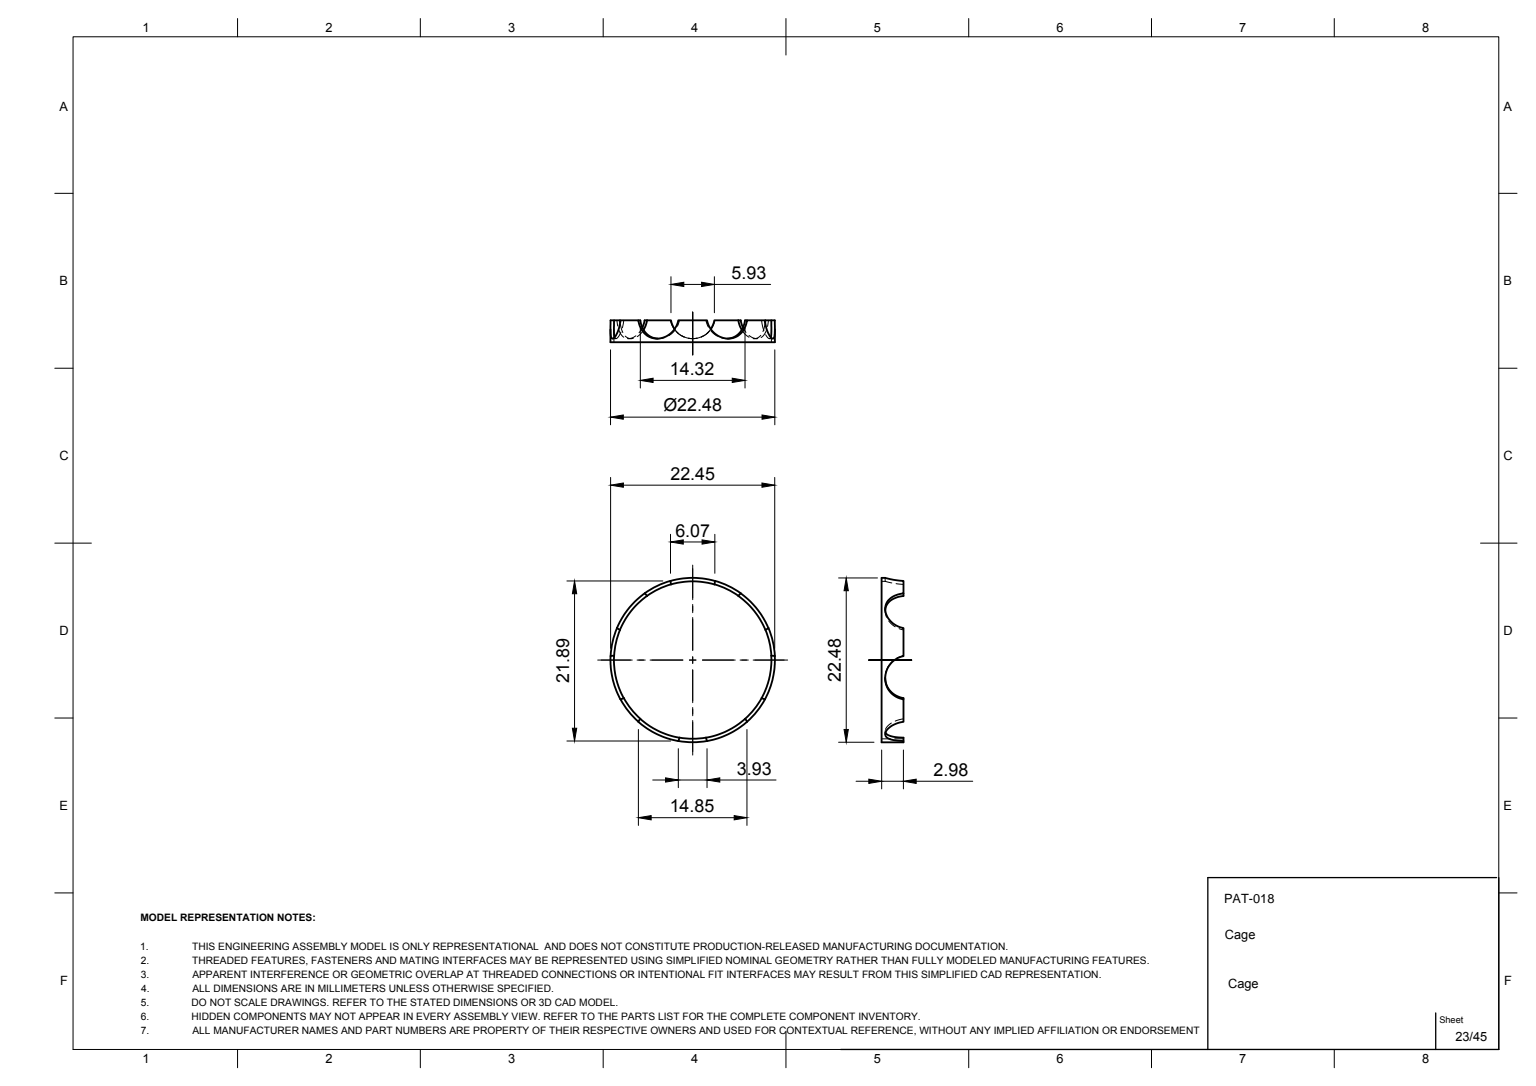
ISO-10303-21;
HEADER;
/* Generated by software containing ST-Developer
 * from STEP Tools, Inc. (www.steptools.com) 
 */

FILE_DESCRIPTION(
/* description */ ('Cam-driven reciprocating slide'),
/* implementation_level */ '2;1');

FILE_NAME(
/* name */ 'Cage.step',
/* time_stamp */ '2026-10-28T03:25:20-07:00',
/* author */ (''),
/* organization */ (''),
/* preprocessor_version */ 'ST-DEVELOPER v20.2',
/* originating_system */ 'Autodesk Translation Framework v15.17.0.0',
/* authorisation */ '');

FILE_SCHEMA (('AUTOMOTIVE_DESIGN { 1 0 10303 214 3 1 1 }'));
ENDSEC;

DATA;
#10=MECHANICAL_DESIGN_GEOMETRIC_PRESENTATION_REPRESENTATION('',(#444),#13277);
#308=SPHERICAL_SURFACE('',#7211,0.309556);
#309=SPHERICAL_SURFACE('',#7227,0.309556);
#310=SPHERICAL_SURFACE('',#7232,0.309556);
#311=SPHERICAL_SURFACE('',#7238,0.309556);
#312=SPHERICAL_SURFACE('',#7243,0.309556);
#313=SPHERICAL_SURFACE('',#7248,0.309556);
#314=SPHERICAL_SURFACE('',#7256,0.309556);
#333=B_SPLINE_CURVE_WITH_KNOTS('',3,(#11932,#11933,#11934,#11935,#11936,
#11937,#11938,#11939,#11940,#11941,#11942,#11943,#11944,#11945,#11946,#11947,
#11948,#11949,#11950,#11951,#11952,#11953),.UNSPECIFIED.,.F.,.F.,(4,2,2,
2,2,2,2,2,2,2,4),(0.0591825211272536,0.157966726598481,0.236950089897721,
0.315933453196962,0.391576304923761,0.46721915665056,0.54286200837736,0.618504860104159,
0.697488223403399,0.77647158670264,0.875255792173867),.UNSPECIFIED.);
#334=B_SPLINE_CURVE_WITH_KNOTS('',3,(#11957,#11958,#11959,#11960,#11961,
#11962,#11963,#11964,#11965,#11966,#11967,#11968,#11969,#11970,#11971,#11972,
#11973,#11974,#11975,#11976,#11977,#11978),.UNSPECIFIED.,.F.,.F.,(4,2,2,
2,2,2,2,2,2,2,4),(0.0581119756758434,0.106553146291161,0.213106292582322,
0.30849933801665,0.386091982889075,0.4636846277615,0.541277272633925,0.61886991750635,
0.714262962940678,0.820816109231839,0.869257279847157),.UNSPECIFIED.);
#335=B_SPLINE_CURVE_WITH_KNOTS('',3,(#11984,#11985,#11986,#11987,#11988,
#11989,#11990,#11991,#11992,#11993,#11994,#11995,#11996,#11997,#11998,#11999,
#12000,#12001,#12002,#12003,#12004,#12005),.UNSPECIFIED.,.F.,.F.,(4,2,2,
2,2,2,2,2,2,2,4),(0.0581119756758434,0.106553146291161,0.213106292582322,
0.30849933801665,0.386091982889075,0.4636846277615,0.541277272633925,0.61886991750635,
0.714262962940679,0.820816109231839,0.869257279847157),.UNSPECIFIED.);
#336=B_SPLINE_CURVE_WITH_KNOTS('',3,(#12009,#12010,#12011,#12012,#12013,
#12014,#12015,#12016,#12017,#12018,#12019,#12020,#12021,#12022,#12023,#12024,
#12025,#12026,#12027,#12028,#12029,#12030),.UNSPECIFIED.,.F.,.F.,(4,2,2,
2,2,2,2,2,2,2,4),(0.0581119756758433,0.106553146291161,0.213106292582322,
0.308499338016649,0.386091982889075,0.4636846277615,0.541277272633925,0.61886991750635,
0.714262962940678,0.820816109231839,0.869257279847157),.UNSPECIFIED.);
#337=B_SPLINE_CURVE_WITH_KNOTS('',3,(#12039,#12040,#12041,#12042,#12043,
#12044,#12045,#12046,#12047,#12048,#12049,#12050,#12051,#12052,#12053,#12054,
#12055,#12056,#12057,#12058,#12059,#12060),.UNSPECIFIED.,.F.,.F.,(4,2,2,
2,2,2,2,2,2,2,4),(0.0581119756758433,0.106553146291161,0.213106292582322,
0.30849933801665,0.386091982889075,0.4636846277615,0.541277272633925,0.61886991750635,
0.714262962940678,0.820816109231839,0.869257279847157),.UNSPECIFIED.);
#338=B_SPLINE_CURVE_WITH_KNOTS('',3,(#12064,#12065,#12066,#12067,#12068,
#12069,#12070,#12071,#12072,#12073,#12074,#12075,#12076,#12077,#12078,#12079,
#12080,#12081,#12082,#12083,#12084,#12085),.UNSPECIFIED.,.F.,.F.,(4,2,2,
2,2,2,2,2,2,2,4),(0.0581119756758434,0.106553146291161,0.213106292582322,
0.30849933801665,0.386091982889075,0.4636846277615,0.541277272633925,0.61886991750635,
0.714262962940678,0.820816109231839,0.869257279847157),.UNSPECIFIED.);
#339=B_SPLINE_CURVE_WITH_KNOTS('',3,(#12089,#12090,#12091,#12092,#12093,
#12094,#12095,#12096,#12097,#12098,#12099,#12100,#12101,#12102,#12103,#12104,
#12105,#12106,#12107,#12108,#12109,#12110),.UNSPECIFIED.,.F.,.F.,(4,2,2,
2,2,2,2,2,2,2,4),(0.0581119756758434,0.106553146291161,0.213106292582322,
0.30849933801665,0.386091982889075,0.4636846277615,0.541277272633925,0.61886991750635,
0.714262962940678,0.820816109231839,0.869257279847157),.UNSPECIFIED.);
#340=B_SPLINE_CURVE_WITH_KNOTS('',3,(#12114,#12115,#12116,#12117,#12118,
#12119,#12120,#12121,#12122,#12123,#12124,#12125,#12126,#12127,#12128,#12129,
#12130,#12131,#12132,#12133,#12134,#12135),.UNSPECIFIED.,.F.,.F.,(4,2,2,
2,2,2,2,2,2,2,4),(0.0581119756758433,0.106553146291161,0.213106292582322,
0.30849933801665,0.386091982889075,0.4636846277615,0.541277272633925,0.61886991750635,
0.714262962940678,0.820816109231839,0.869257279847157),.UNSPECIFIED.);
#341=B_SPLINE_CURVE_WITH_KNOTS('',3,(#12143,#12144,#12145,#12146,#12147,
#12148,#12149,#12150,#12151,#12152,#12153,#12154,#12155,#12156,#12157,#12158,
#12159,#12160,#12161,#12162,#12163,#12164),.UNSPECIFIED.,.F.,.F.,(4,2,2,
2,2,2,2,2,2,2,4),(0.0591825211272536,0.157966726598481,0.236950089897721,
0.315933453196962,0.391576304923761,0.467219156650561,0.54286200837736,
0.618504860104159,0.697488223403399,0.77647158670264,0.875255792173867),
 .UNSPECIFIED.);
#342=B_SPLINE_CURVE_WITH_KNOTS('',3,(#12172,#12173,#12174,#12175,#12176,
#12177,#12178,#12179,#12180,#12181,#12182,#12183,#12184,#12185,#12186,#12187,
#12188,#12189,#12190,#12191,#12192,#12193),.UNSPECIFIED.,.F.,.F.,(4,2,2,
2,2,2,2,2,2,2,4),(0.0591825211272536,0.157966726598481,0.236950089897722,
0.315933453196962,0.391576304923761,0.467219156650561,0.54286200837736,
0.618504860104159,0.697488223403399,0.77647158670264,0.875255792173867),
 .UNSPECIFIED.);
#343=B_SPLINE_CURVE_WITH_KNOTS('',3,(#12203,#12204,#12205,#12206,#12207,
#12208,#12209,#12210,#12211,#12212,#12213,#12214,#12215,#12216,#12217,#12218,
#12219,#12220,#12221,#12222,#12223,#12224),.UNSPECIFIED.,.F.,.F.,(4,2,2,
2,2,2,2,2,2,2,4),(0.0591825211272536,0.157966726598481,0.236950089897721,
0.315933453196962,0.391576304923761,0.46721915665056,0.54286200837736,0.618504860104159,
0.697488223403399,0.77647158670264,0.875255792173867),.UNSPECIFIED.);
#344=B_SPLINE_CURVE_WITH_KNOTS('',3,(#12232,#12233,#12234,#12235,#12236,
#12237,#12238,#12239,#12240,#12241,#12242,#12243,#12244,#12245,#12246,#12247,
#12248,#12249,#12250,#12251,#12252,#12253),.UNSPECIFIED.,.F.,.F.,(4,2,2,
2,2,2,2,2,2,2,4),(0.0591825211272536,0.157966726598481,0.236950089897721,
0.315933453196962,0.391576304923761,0.46721915665056,0.542862008377359,
0.618504860104159,0.697488223403399,0.776471586702639,0.875255792173867),
 .UNSPECIFIED.);
#345=B_SPLINE_CURVE_WITH_KNOTS('',3,(#12261,#12262,#12263,#12264,#12265,
#12266,#12267,#12268,#12269,#12270,#12271,#12272,#12273,#12274,#12275,#12276,
#12277,#12278,#12279,#12280,#12281,#12282),.UNSPECIFIED.,.F.,.F.,(4,2,2,
2,2,2,2,2,2,2,4),(0.0591825211272536,0.157966726598481,0.236950089897721,
0.315933453196962,0.391576304923761,0.46721915665056,0.54286200837736,0.618504860104159,
0.697488223403399,0.77647158670264,0.875255792173867),.UNSPECIFIED.);
#346=B_SPLINE_CURVE_WITH_KNOTS('',3,(#12291,#12292,#12293,#12294,#12295,
#12296,#12297,#12298,#12299,#12300,#12301,#12302,#12303,#12304,#12305,#12306,
#12307,#12308,#12309,#12310,#12311,#12312),.UNSPECIFIED.,.F.,.F.,(4,2,2,
2,2,2,2,2,2,2,4),(0.0591825211272536,0.157966726598481,0.236950089897721,
0.315933453196962,0.391576304923761,0.46721915665056,0.542862008377359,
0.618504860104159,0.697488223403399,0.776471586702639,0.875255792173867),
 .UNSPECIFIED.);
#364=SHAPE_REPRESENTATION_RELATIONSHIP('SRR','None',#13458,#401);
#401=ADVANCED_BREP_SHAPE_REPRESENTATION('',(#488),#13253);
#444=STYLED_ITEM('',(#13720),#488);
#488=MANIFOLD_SOLID_BREP('Continuous crown cage',#6420);
#622=FACE_BOUND('',#1585,.T.);
#768=PLANE('',#7224);
#769=PLANE('',#7229);
#770=PLANE('',#7234);
#771=PLANE('',#7240);
#772=PLANE('',#7245);
#773=PLANE('',#7254);
#774=PLANE('',#7258);
#775=PLANE('',#7259);
#1075=FACE_OUTER_BOUND('',#1569,.T.);
#1076=FACE_OUTER_BOUND('',#1570,.T.);
#1077=FACE_OUTER_BOUND('',#1571,.T.);
#1078=FACE_OUTER_BOUND('',#1572,.T.);
#1079=FACE_OUTER_BOUND('',#1573,.T.);
#1080=FACE_OUTER_BOUND('',#1574,.T.);
#1081=FACE_OUTER_BOUND('',#1575,.T.);
#1082=FACE_OUTER_BOUND('',#1576,.T.);
#1083=FACE_OUTER_BOUND('',#1577,.T.);
#1084=FACE_OUTER_BOUND('',#1578,.T.);
#1085=FACE_OUTER_BOUND('',#1579,.T.);
#1086=FACE_OUTER_BOUND('',#1580,.T.);
#1087=FACE_OUTER_BOUND('',#1581,.T.);
#1088=FACE_OUTER_BOUND('',#1582,.T.);
#1089=FACE_OUTER_BOUND('',#1583,.T.);
#1090=FACE_OUTER_BOUND('',#1584,.T.);
#1091=FACE_OUTER_BOUND('',#1586,.T.);
#1569=EDGE_LOOP('',(#5086,#5087,#5088,#5089));
#1570=EDGE_LOOP('',(#5090,#5091,#5092,#5093,#5094,#5095,#5096,#5097,#5098,
#5099,#5100,#5101,#5102,#5103,#5104,#5105,#5106,#5107));
#1571=EDGE_LOOP('',(#5108,#5109,#5110,#5111));
#1572=EDGE_LOOP('',(#5112,#5113,#5114,#5115));
#1573=EDGE_LOOP('',(#5116,#5117,#5118,#5119));
#1574=EDGE_LOOP('',(#5120,#5121,#5122,#5123));
#1575=EDGE_LOOP('',(#5124,#5125,#5126,#5127,#5128,#5129));
#1576=EDGE_LOOP('',(#5130,#5131,#5132,#5133));
#1577=EDGE_LOOP('',(#5134,#5135,#5136,#5137));
#1578=EDGE_LOOP('',(#5138,#5139,#5140,#5141));
#1579=EDGE_LOOP('',(#5142,#5143,#5144,#5145));
#1580=EDGE_LOOP('',(#5146,#5147,#5148,#5149));
#1581=EDGE_LOOP('',(#5150,#5151,#5152,#5153,#5154,#5155,#5156,#5157,#5158,
#5159,#5160,#5161,#5162,#5163,#5164,#5165,#5166,#5167));
#1582=EDGE_LOOP('',(#5168,#5169,#5170,#5171));
#1583=EDGE_LOOP('',(#5172,#5173,#5174,#5175));
#1584=EDGE_LOOP('',(#5176));
#1585=EDGE_LOOP('',(#5177));
#1586=EDGE_LOOP('',(#5178,#5179,#5180,#5181));
#2042=LINE('',#12034,#2481);
#2043=LINE('',#12287,#2482);
#2481=VECTOR('',#8608,1.123812);
#2482=VECTOR('',#8677,1.076188);
#2876=CIRCLE('',#7212,0.303778037777585);
#2877=CIRCLE('',#7213,0.303778037777585);
#2878=CIRCLE('',#7215,1.123812);
#2879=CIRCLE('',#7216,1.123812);
#2880=CIRCLE('',#7217,1.123812);
#2881=CIRCLE('',#7218,1.123812);
#2882=CIRCLE('',#7219,1.123812);
#2883=CIRCLE('',#7220,1.123812);
#2884=CIRCLE('',#7221,1.123812);
#2885=CIRCLE('',#7222,1.123812);
#2886=CIRCLE('',#7223,1.123812);
#2887=CIRCLE('',#7225,1.076188);
#2888=CIRCLE('',#7226,0.303778037777585);
#2889=CIRCLE('',#7228,0.303778037777585);
#2890=CIRCLE('',#7230,1.076188);
#2891=CIRCLE('',#7231,0.303778037777585);
#2892=CIRCLE('',#7233,0.303778037777585);
#2893=CIRCLE('',#7235,1.076188);
#2894=CIRCLE('',#7236,1.076188);
#2895=CIRCLE('',#7237,0.303778037777585);
#2896=CIRCLE('',#7239,0.303778037777585);
#2897=CIRCLE('',#7241,1.076188);
#2898=CIRCLE('',#7242,0.303778037777585);
#2899=CIRCLE('',#7244,0.303778037777585);
#2900=CIRCLE('',#7246,1.076188);
#2901=CIRCLE('',#7247,0.303778037777585);
#2902=CIRCLE('',#7249,0.303778037777585);
#2903=CIRCLE('',#7251,1.076188);
#2904=CIRCLE('',#7252,1.076188);
#2905=CIRCLE('',#7253,1.076188);
#2906=CIRCLE('',#7255,0.303778037777585);
#2907=CIRCLE('',#7257,0.303778037777585);
#3293=VERTEX_POINT('',#11930);
#3294=VERTEX_POINT('',#11931);
#3295=VERTEX_POINT('',#11954);
#3296=VERTEX_POINT('',#11956);
#3297=VERTEX_POINT('',#11981);
#3298=VERTEX_POINT('',#11983);
#3299=VERTEX_POINT('',#12006);
#3300=VERTEX_POINT('',#12008);
#3301=VERTEX_POINT('',#12031);
#3302=VERTEX_POINT('',#12033);
#3303=VERTEX_POINT('',#12036);
#3304=VERTEX_POINT('',#12038);
#3305=VERTEX_POINT('',#12061);
#3306=VERTEX_POINT('',#12063);
#3307=VERTEX_POINT('',#12086);
#3308=VERTEX_POINT('',#12088);
#3309=VERTEX_POINT('',#12111);
#3310=VERTEX_POINT('',#12113);
#3311=VERTEX_POINT('',#12138);
#3312=VERTEX_POINT('',#12142);
#3313=VERTEX_POINT('',#12167);
#3314=VERTEX_POINT('',#12171);
#3315=VERTEX_POINT('',#12196);
#3316=VERTEX_POINT('',#12198);
#3317=VERTEX_POINT('',#12202);
#3318=VERTEX_POINT('',#12227);
#3319=VERTEX_POINT('',#12231);
#3320=VERTEX_POINT('',#12256);
#3321=VERTEX_POINT('',#12260);
#3322=VERTEX_POINT('',#12285);
#3323=VERTEX_POINT('',#12288);
#3324=VERTEX_POINT('',#12290);
#3933=EDGE_CURVE('',#3293,#3294,#333,.T.);
#3934=EDGE_CURVE('',#3295,#3293,#2876,.T.);
#3935=EDGE_CURVE('',#3296,#3295,#334,.T.);
#3936=EDGE_CURVE('',#3294,#3296,#2877,.T.);
#3937=EDGE_CURVE('',#3297,#3295,#2878,.T.);
#3938=EDGE_CURVE('',#3297,#3298,#335,.T.);
#3939=EDGE_CURVE('',#3299,#3298,#2879,.T.);
#3940=EDGE_CURVE('',#3299,#3300,#336,.T.);
#3941=EDGE_CURVE('',#3301,#3300,#2880,.T.);
#3942=EDGE_CURVE('',#3301,#3302,#2042,.T.);
#3943=EDGE_CURVE('',#3302,#3302,#2881,.T.);
#3944=EDGE_CURVE('',#3303,#3301,#2882,.T.);
#3945=EDGE_CURVE('',#3303,#3304,#337,.T.);
#3946=EDGE_CURVE('',#3305,#3304,#2883,.T.);
#3947=EDGE_CURVE('',#3305,#3306,#338,.T.);
#3948=EDGE_CURVE('',#3307,#3306,#2884,.T.);
#3949=EDGE_CURVE('',#3307,#3308,#339,.T.);
#3950=EDGE_CURVE('',#3309,#3308,#2885,.T.);
#3951=EDGE_CURVE('',#3309,#3310,#340,.T.);
#3952=EDGE_CURVE('',#3296,#3310,#2886,.T.);
#3953=EDGE_CURVE('',#3293,#3311,#2887,.T.);
#3954=EDGE_CURVE('',#3311,#3297,#2888,.T.);
#3955=EDGE_CURVE('',#3312,#3311,#341,.T.);
#3956=EDGE_CURVE('',#3298,#3312,#2889,.T.);
#3957=EDGE_CURVE('',#3312,#3313,#2890,.T.);
#3958=EDGE_CURVE('',#3313,#3299,#2891,.T.);
#3959=EDGE_CURVE('',#3314,#3313,#342,.T.);
#3960=EDGE_CURVE('',#3300,#3314,#2892,.T.);
#3961=EDGE_CURVE('',#3314,#3315,#2893,.T.);
#3962=EDGE_CURVE('',#3315,#3316,#2894,.T.);
#3963=EDGE_CURVE('',#3316,#3303,#2895,.T.);
#3964=EDGE_CURVE('',#3317,#3316,#343,.T.);
#3965=EDGE_CURVE('',#3304,#3317,#2896,.T.);
#3966=EDGE_CURVE('',#3317,#3318,#2897,.T.);
#3967=EDGE_CURVE('',#3318,#3305,#2898,.T.);
#3968=EDGE_CURVE('',#3319,#3318,#344,.T.);
#3969=EDGE_CURVE('',#3306,#3319,#2899,.T.);
#3970=EDGE_CURVE('',#3319,#3320,#2900,.T.);
#3971=EDGE_CURVE('',#3320,#3307,#2901,.T.);
#3972=EDGE_CURVE('',#3321,#3320,#345,.T.);
#3973=EDGE_CURVE('',#3308,#3321,#2902,.T.);
#3974=EDGE_CURVE('',#3322,#3322,#2903,.T.);
#3975=EDGE_CURVE('',#3322,#3315,#2043,.T.);
#3976=EDGE_CURVE('',#3323,#3294,#2904,.T.);
#3977=EDGE_CURVE('',#3323,#3324,#346,.T.);
#3978=EDGE_CURVE('',#3321,#3324,#2905,.T.);
#3979=EDGE_CURVE('',#3310,#3323,#2906,.T.);
#3980=EDGE_CURVE('',#3324,#3309,#2907,.T.);
#5086=ORIENTED_EDGE('',*,*,#3933,.F.);
#5087=ORIENTED_EDGE('',*,*,#3934,.F.);
#5088=ORIENTED_EDGE('',*,*,#3935,.F.);
#5089=ORIENTED_EDGE('',*,*,#3936,.F.);
#5090=ORIENTED_EDGE('',*,*,#3935,.T.);
#5091=ORIENTED_EDGE('',*,*,#3937,.F.);
#5092=ORIENTED_EDGE('',*,*,#3938,.T.);
#5093=ORIENTED_EDGE('',*,*,#3939,.F.);
#5094=ORIENTED_EDGE('',*,*,#3940,.T.);
#5095=ORIENTED_EDGE('',*,*,#3941,.F.);
#5096=ORIENTED_EDGE('',*,*,#3942,.T.);
#5097=ORIENTED_EDGE('',*,*,#3943,.F.);
#5098=ORIENTED_EDGE('',*,*,#3942,.F.);
#5099=ORIENTED_EDGE('',*,*,#3944,.F.);
#5100=ORIENTED_EDGE('',*,*,#3945,.T.);
#5101=ORIENTED_EDGE('',*,*,#3946,.F.);
#5102=ORIENTED_EDGE('',*,*,#3947,.T.);
#5103=ORIENTED_EDGE('',*,*,#3948,.F.);
#5104=ORIENTED_EDGE('',*,*,#3949,.T.);
#5105=ORIENTED_EDGE('',*,*,#3950,.F.);
#5106=ORIENTED_EDGE('',*,*,#3951,.T.);
#5107=ORIENTED_EDGE('',*,*,#3952,.F.);
#5108=ORIENTED_EDGE('',*,*,#3934,.T.);
#5109=ORIENTED_EDGE('',*,*,#3953,.T.);
#5110=ORIENTED_EDGE('',*,*,#3954,.T.);
#5111=ORIENTED_EDGE('',*,*,#3937,.T.);
#5112=ORIENTED_EDGE('',*,*,#3955,.F.);
#5113=ORIENTED_EDGE('',*,*,#3956,.F.);
#5114=ORIENTED_EDGE('',*,*,#3938,.F.);
#5115=ORIENTED_EDGE('',*,*,#3954,.F.);
#5116=ORIENTED_EDGE('',*,*,#3956,.T.);
#5117=ORIENTED_EDGE('',*,*,#3957,.T.);
#5118=ORIENTED_EDGE('',*,*,#3958,.T.);
#5119=ORIENTED_EDGE('',*,*,#3939,.T.);
#5120=ORIENTED_EDGE('',*,*,#3959,.F.);
#5121=ORIENTED_EDGE('',*,*,#3960,.F.);
#5122=ORIENTED_EDGE('',*,*,#3940,.F.);
#5123=ORIENTED_EDGE('',*,*,#3958,.F.);
#5124=ORIENTED_EDGE('',*,*,#3960,.T.);
#5125=ORIENTED_EDGE('',*,*,#3961,.T.);
#5126=ORIENTED_EDGE('',*,*,#3962,.T.);
#5127=ORIENTED_EDGE('',*,*,#3963,.T.);
#5128=ORIENTED_EDGE('',*,*,#3944,.T.);
#5129=ORIENTED_EDGE('',*,*,#3941,.T.);
#5130=ORIENTED_EDGE('',*,*,#3964,.F.);
#5131=ORIENTED_EDGE('',*,*,#3965,.F.);
#5132=ORIENTED_EDGE('',*,*,#3945,.F.);
#5133=ORIENTED_EDGE('',*,*,#3963,.F.);
#5134=ORIENTED_EDGE('',*,*,#3965,.T.);
#5135=ORIENTED_EDGE('',*,*,#3966,.T.);
#5136=ORIENTED_EDGE('',*,*,#3967,.T.);
#5137=ORIENTED_EDGE('',*,*,#3946,.T.);
#5138=ORIENTED_EDGE('',*,*,#3968,.F.);
#5139=ORIENTED_EDGE('',*,*,#3969,.F.);
#5140=ORIENTED_EDGE('',*,*,#3947,.F.);
#5141=ORIENTED_EDGE('',*,*,#3967,.F.);
#5142=ORIENTED_EDGE('',*,*,#3969,.T.);
#5143=ORIENTED_EDGE('',*,*,#3970,.T.);
#5144=ORIENTED_EDGE('',*,*,#3971,.T.);
#5145=ORIENTED_EDGE('',*,*,#3948,.T.);
#5146=ORIENTED_EDGE('',*,*,#3949,.F.);
#5147=ORIENTED_EDGE('',*,*,#3971,.F.);
#5148=ORIENTED_EDGE('',*,*,#3972,.F.);
#5149=ORIENTED_EDGE('',*,*,#3973,.F.);
#5150=ORIENTED_EDGE('',*,*,#3974,.F.);
#5151=ORIENTED_EDGE('',*,*,#3975,.T.);
#5152=ORIENTED_EDGE('',*,*,#3961,.F.);
#5153=ORIENTED_EDGE('',*,*,#3959,.T.);
#5154=ORIENTED_EDGE('',*,*,#3957,.F.);
#5155=ORIENTED_EDGE('',*,*,#3955,.T.);
#5156=ORIENTED_EDGE('',*,*,#3953,.F.);
#5157=ORIENTED_EDGE('',*,*,#3933,.T.);
#5158=ORIENTED_EDGE('',*,*,#3976,.F.);
#5159=ORIENTED_EDGE('',*,*,#3977,.T.);
#5160=ORIENTED_EDGE('',*,*,#3978,.F.);
#5161=ORIENTED_EDGE('',*,*,#3972,.T.);
#5162=ORIENTED_EDGE('',*,*,#3970,.F.);
#5163=ORIENTED_EDGE('',*,*,#3968,.T.);
#5164=ORIENTED_EDGE('',*,*,#3966,.F.);
#5165=ORIENTED_EDGE('',*,*,#3964,.T.);
#5166=ORIENTED_EDGE('',*,*,#3962,.F.);
#5167=ORIENTED_EDGE('',*,*,#3975,.F.);
#5168=ORIENTED_EDGE('',*,*,#3936,.T.);
#5169=ORIENTED_EDGE('',*,*,#3952,.T.);
#5170=ORIENTED_EDGE('',*,*,#3979,.T.);
#5171=ORIENTED_EDGE('',*,*,#3976,.T.);
#5172=ORIENTED_EDGE('',*,*,#3951,.F.);
#5173=ORIENTED_EDGE('',*,*,#3980,.F.);
#5174=ORIENTED_EDGE('',*,*,#3977,.F.);
#5175=ORIENTED_EDGE('',*,*,#3979,.F.);
#5176=ORIENTED_EDGE('',*,*,#3943,.T.);
#5177=ORIENTED_EDGE('',*,*,#3974,.T.);
#5178=ORIENTED_EDGE('',*,*,#3973,.T.);
#5179=ORIENTED_EDGE('',*,*,#3978,.T.);
#5180=ORIENTED_EDGE('',*,*,#3980,.T.);
#5181=ORIENTED_EDGE('',*,*,#3950,.T.);
#5965=CYLINDRICAL_SURFACE('',#7214,1.123812);
#5966=CYLINDRICAL_SURFACE('',#7250,1.076188);
#6193=ADVANCED_FACE('',(#1075),#308,.F.);
#6194=ADVANCED_FACE('',(#1076),#5965,.T.);
#6195=ADVANCED_FACE('',(#1077),#768,.T.);
#6196=ADVANCED_FACE('',(#1078),#309,.F.);
#6197=ADVANCED_FACE('',(#1079),#769,.T.);
#6198=ADVANCED_FACE('',(#1080),#310,.F.);
#6199=ADVANCED_FACE('',(#1081),#770,.T.);
#6200=ADVANCED_FACE('',(#1082),#311,.F.);
#6201=ADVANCED_FACE('',(#1083),#771,.T.);
#6202=ADVANCED_FACE('',(#1084),#312,.F.);
#6203=ADVANCED_FACE('',(#1085),#772,.T.);
#6204=ADVANCED_FACE('',(#1086),#313,.F.);
#6205=ADVANCED_FACE('',(#1087),#5966,.F.);
#6206=ADVANCED_FACE('',(#1088),#773,.T.);
#6207=ADVANCED_FACE('',(#1089),#314,.F.);
#6208=ADVANCED_FACE('',(#1090,#622),#774,.T.);
#6209=ADVANCED_FACE('',(#1091),#775,.T.);
#6420=CLOSED_SHELL('',(#6193,#6194,#6195,#6196,#6197,#6198,#6199,#6200,
#6201,#6202,#6203,#6204,#6205,#6206,#6207,#6208,#6209));
#7210=AXIS2_PLACEMENT_3D('',#11928,#8592,#8593);
#7211=AXIS2_PLACEMENT_3D('',#11929,#8594,#8595);
#7212=AXIS2_PLACEMENT_3D('',#11955,#8596,#8597);
#7213=AXIS2_PLACEMENT_3D('',#11979,#8598,#8599);
#7214=AXIS2_PLACEMENT_3D('',#11980,#8600,#8601);
#7215=AXIS2_PLACEMENT_3D('',#11982,#8602,#8603);
#7216=AXIS2_PLACEMENT_3D('',#12007,#8604,#8605);
#7217=AXIS2_PLACEMENT_3D('',#12032,#8606,#8607);
#7218=AXIS2_PLACEMENT_3D('',#12035,#8609,#8610);
#7219=AXIS2_PLACEMENT_3D('',#12037,#8611,#8612);
#7220=AXIS2_PLACEMENT_3D('',#12062,#8613,#8614);
#7221=AXIS2_PLACEMENT_3D('',#12087,#8615,#8616);
#7222=AXIS2_PLACEMENT_3D('',#12112,#8617,#8618);
#7223=AXIS2_PLACEMENT_3D('',#12136,#8619,#8620);
#7224=AXIS2_PLACEMENT_3D('',#12137,#8621,#8622);
#7225=AXIS2_PLACEMENT_3D('',#12139,#8623,#8624);
#7226=AXIS2_PLACEMENT_3D('',#12140,#8625,#8626);
#7227=AXIS2_PLACEMENT_3D('',#12141,#8627,#8628);
#7228=AXIS2_PLACEMENT_3D('',#12165,#8629,#8630);
#7229=AXIS2_PLACEMENT_3D('',#12166,#8631,#8632);
#7230=AXIS2_PLACEMENT_3D('',#12168,#8633,#8634);
#7231=AXIS2_PLACEMENT_3D('',#12169,#8635,#8636);
#7232=AXIS2_PLACEMENT_3D('',#12170,#8637,#8638);
#7233=AXIS2_PLACEMENT_3D('',#12194,#8639,#8640);
#7234=AXIS2_PLACEMENT_3D('',#12195,#8641,#8642);
#7235=AXIS2_PLACEMENT_3D('',#12197,#8643,#8644);
#7236=AXIS2_PLACEMENT_3D('',#12199,#8645,#8646);
#7237=AXIS2_PLACEMENT_3D('',#12200,#8647,#8648);
#7238=AXIS2_PLACEMENT_3D('',#12201,#8649,#8650);
#7239=AXIS2_PLACEMENT_3D('',#12225,#8651,#8652);
#7240=AXIS2_PLACEMENT_3D('',#12226,#8653,#8654);
#7241=AXIS2_PLACEMENT_3D('',#12228,#8655,#8656);
#7242=AXIS2_PLACEMENT_3D('',#12229,#8657,#8658);
#7243=AXIS2_PLACEMENT_3D('',#12230,#8659,#8660);
#7244=AXIS2_PLACEMENT_3D('',#12254,#8661,#8662);
#7245=AXIS2_PLACEMENT_3D('',#12255,#8663,#8664);
#7246=AXIS2_PLACEMENT_3D('',#12257,#8665,#8666);
#7247=AXIS2_PLACEMENT_3D('',#12258,#8667,#8668);
#7248=AXIS2_PLACEMENT_3D('',#12259,#8669,#8670);
#7249=AXIS2_PLACEMENT_3D('',#12283,#8671,#8672);
#7250=AXIS2_PLACEMENT_3D('',#12284,#8673,#8674);
#7251=AXIS2_PLACEMENT_3D('',#12286,#8675,#8676);
#7252=AXIS2_PLACEMENT_3D('',#12289,#8678,#8679);
#7253=AXIS2_PLACEMENT_3D('',#12313,#8680,#8681);
#7254=AXIS2_PLACEMENT_3D('',#12314,#8682,#8683);
#7255=AXIS2_PLACEMENT_3D('',#12315,#8684,#8685);
#7256=AXIS2_PLACEMENT_3D('',#12316,#8686,#8687);
#7257=AXIS2_PLACEMENT_3D('',#12317,#8688,#8689);
#7258=AXIS2_PLACEMENT_3D('',#12318,#8690,#8691);
#7259=AXIS2_PLACEMENT_3D('',#12319,#8692,#8693);
#8592=DIRECTION('axis',(0.,0.,1.));
#8593=DIRECTION('refdir',(1.,0.,0.));
#8594=DIRECTION('center_axis',(0.,0.,1.));
#8595=DIRECTION('ref_axis',(1.,0.,0.));
#8596=DIRECTION('center_axis',(0.,-1.,0.));
#8597=DIRECTION('ref_axis',(0.,0.,-1.));
#8598=DIRECTION('center_axis',(0.,-1.,0.));
#8599=DIRECTION('ref_axis',(0.,0.,-1.));
#8600=DIRECTION('center_axis',(0.,1.,0.));
#8601=DIRECTION('ref_axis',(1.,0.,0.));
#8602=DIRECTION('center_axis',(0.,1.,0.));
#8603=DIRECTION('ref_axis',(1.,0.,0.));
#8604=DIRECTION('center_axis',(0.,1.,0.));
#8605=DIRECTION('ref_axis',(1.,0.,0.));
#8606=DIRECTION('center_axis',(0.,1.,0.));
#8607=DIRECTION('ref_axis',(1.,0.,0.));
#8608=DIRECTION('',(0.,-1.,0.));
#8609=DIRECTION('center_axis',(0.,-1.,0.));
#8610=DIRECTION('ref_axis',(1.,0.,0.));
#8611=DIRECTION('center_axis',(0.,1.,0.));
#8612=DIRECTION('ref_axis',(1.,0.,0.));
#8613=DIRECTION('center_axis',(0.,1.,0.));
#8614=DIRECTION('ref_axis',(1.,0.,0.));
#8615=DIRECTION('center_axis',(0.,1.,0.));
#8616=DIRECTION('ref_axis',(1.,0.,0.));
#8617=DIRECTION('center_axis',(0.,1.,0.));
#8618=DIRECTION('ref_axis',(1.,0.,0.));
#8619=DIRECTION('center_axis',(0.,1.,0.));
#8620=DIRECTION('ref_axis',(1.,0.,0.));
#8621=DIRECTION('center_axis',(0.,1.,0.));
#8622=DIRECTION('ref_axis',(1.,0.,0.));
#8623=DIRECTION('center_axis',(0.,-1.,0.));
#8624=DIRECTION('ref_axis',(1.,0.,0.));
#8625=DIRECTION('center_axis',(0.,-1.,0.));
#8626=DIRECTION('ref_axis',(0.,0.,-1.));
#8627=DIRECTION('center_axis',(8.96625347776458E-17,0.,1.));
#8628=DIRECTION('ref_axis',(1.,0.,0.));
#8629=DIRECTION('center_axis',(0.,-1.,0.));
#8630=DIRECTION('ref_axis',(0.,0.,-1.));
#8631=DIRECTION('center_axis',(0.,1.,0.));
#8632=DIRECTION('ref_axis',(1.,0.,0.));
#8633=DIRECTION('center_axis',(0.,-1.,0.));
#8634=DIRECTION('ref_axis',(1.,0.,0.));
#8635=DIRECTION('center_axis',(0.,-1.,0.));
#8636=DIRECTION('ref_axis',(0.,0.,-1.));
#8637=DIRECTION('center_axis',(0.,0.,1.));
#8638=DIRECTION('ref_axis',(1.,0.,0.));
#8639=DIRECTION('center_axis',(0.,-1.,0.));
#8640=DIRECTION('ref_axis',(0.,0.,-1.));
#8641=DIRECTION('center_axis',(0.,1.,0.));
#8642=DIRECTION('ref_axis',(1.,0.,0.));
#8643=DIRECTION('center_axis',(0.,-1.,0.));
#8644=DIRECTION('ref_axis',(1.,0.,0.));
#8645=DIRECTION('center_axis',(0.,-1.,0.));
#8646=DIRECTION('ref_axis',(1.,0.,0.));
#8647=DIRECTION('center_axis',(0.,-1.,0.));
#8648=DIRECTION('ref_axis',(0.,0.,-1.));
#8649=DIRECTION('center_axis',(0.,0.,1.));
#8650=DIRECTION('ref_axis',(1.,0.,0.));
#8651=DIRECTION('center_axis',(0.,-1.,0.));
#8652=DIRECTION('ref_axis',(0.,0.,-1.));
#8653=DIRECTION('center_axis',(0.,1.,0.));
#8654=DIRECTION('ref_axis',(1.,0.,0.));
#8655=DIRECTION('center_axis',(0.,-1.,0.));
#8656=DIRECTION('ref_axis',(1.,0.,0.));
#8657=DIRECTION('center_axis',(0.,-1.,0.));
#8658=DIRECTION('ref_axis',(0.,0.,-1.));
#8659=DIRECTION('center_axis',(8.96625347776458E-17,0.,1.));
#8660=DIRECTION('ref_axis',(1.,0.,0.));
#8661=DIRECTION('center_axis',(0.,-1.,0.));
#8662=DIRECTION('ref_axis',(0.,0.,-1.));
#8663=DIRECTION('center_axis',(0.,1.,0.));
#8664=DIRECTION('ref_axis',(1.,0.,0.));
#8665=DIRECTION('center_axis',(0.,-1.,0.));
#8666=DIRECTION('ref_axis',(1.,0.,0.));
#8667=DIRECTION('center_axis',(0.,-1.,0.));
#8668=DIRECTION('ref_axis',(0.,0.,-1.));
#8669=DIRECTION('center_axis',(0.,0.,1.));
#8670=DIRECTION('ref_axis',(1.,0.,0.));
#8671=DIRECTION('center_axis',(0.,-1.,0.));
#8672=DIRECTION('ref_axis',(0.,0.,-1.));
#8673=DIRECTION('center_axis',(0.,1.,0.));
#8674=DIRECTION('ref_axis',(1.,0.,0.));
#8675=DIRECTION('center_axis',(0.,1.,0.));
#8676=DIRECTION('ref_axis',(1.,0.,0.));
#8677=DIRECTION('',(0.,1.,0.));
#8678=DIRECTION('center_axis',(0.,-1.,0.));
#8679=DIRECTION('ref_axis',(1.,0.,0.));
#8680=DIRECTION('center_axis',(0.,-1.,0.));
#8681=DIRECTION('ref_axis',(1.,0.,0.));
#8682=DIRECTION('center_axis',(0.,1.,0.));
#8683=DIRECTION('ref_axis',(1.,0.,0.));
#8684=DIRECTION('center_axis',(0.,-1.,0.));
#8685=DIRECTION('ref_axis',(0.,0.,-1.));
#8686=DIRECTION('center_axis',(0.,0.,1.));
#8687=DIRECTION('ref_axis',(1.,0.,0.));
#8688=DIRECTION('center_axis',(0.,-1.,0.));
#8689=DIRECTION('ref_axis',(0.,0.,-1.));
#8690=DIRECTION('center_axis',(0.,-1.,0.));
#8691=DIRECTION('ref_axis',(-1.,0.,0.));
#8692=DIRECTION('center_axis',(0.,1.,0.));
#8693=DIRECTION('ref_axis',(1.,0.,0.));
#11928=CARTESIAN_POINT('',(0.,0.,0.));
#11929=CARTESIAN_POINT('Origin',(0.685838782044607,0.,0.860014630714833));
#11930=CARTESIAN_POINT('',(0.413083465285518,-0.05953,0.993751811093549));
#11931=CARTESIAN_POINT('',(0.876916659919095,-0.05953,0.623857181492959));
#11932=CARTESIAN_POINT('Ctrl Pts',(0.413083465285518,-0.05953,0.993751811093549));
#11933=CARTESIAN_POINT('Ctrl Pts',(0.419070565453383,-0.0925528133349865,
0.991263089003441));
#11934=CARTESIAN_POINT('Ctrl Pts',(0.430199341854858,-0.124911173756694,
0.986608710139579));
#11935=CARTESIAN_POINT('Ctrl Pts',(0.457978755888596,-0.177924977804098,
0.973971221090534));
#11936=CARTESIAN_POINT('Ctrl Pts',(0.473077587363685,-0.199697230012983,
0.966820759530997));
#11937=CARTESIAN_POINT('Ctrl Pts',(0.507057380724533,-0.237895043532788,
0.949440676105255));
#11938=CARTESIAN_POINT('Ctrl Pts',(0.525933334162555,-0.254319232363049,
0.939198248544428));
#11939=CARTESIAN_POINT('Ctrl Pts',(0.564362943424238,-0.28018331644634,
0.916597376014514));
#11940=CARTESIAN_POINT('Ctrl Pts',(0.585840553788742,-0.29104845371857,
0.903141581680914));
#11941=CARTESIAN_POINT('Ctrl Pts',(0.629305439856167,-0.30527573347708,
0.873412008702649));
#11942=CARTESIAN_POINT('Ctrl Pts',(0.651278921914856,-0.308638795020976,
0.857118508332695));
#11943=CARTESIAN_POINT('Ctrl Pts',(0.690705563850638,-0.308638795020976,
0.825676810575914));
#11944=CARTESIAN_POINT('Ctrl Pts',(0.711480111898423,-0.30527573347708,
0.807879894508811));
#11945=CARTESIAN_POINT('Ctrl Pts',(0.750136149454208,-0.29104845371857,
0.772120216227122));
#11946=CARTESIAN_POINT('Ctrl Pts',(0.768033796848072,-0.28018331644634,
0.754175290318038));
#11947=CARTESIAN_POINT('Ctrl Pts',(0.798619410861634,-0.254319232363049,
0.721738358858166));
#11948=CARTESIAN_POINT('Ctrl Pts',(0.812805334167529,-0.237895043532788,
0.705614819529209));
#11949=CARTESIAN_POINT('Ctrl Pts',(0.837310877969633,-0.199697230012983,
0.676354402927683));
#11950=CARTESIAN_POINT('Ctrl Pts',(0.847641868610495,-0.177924977804098,
0.663225258065736));
#11951=CARTESIAN_POINT('Ctrl Pts',(0.866144010579847,-0.124911173756694,
0.638954437806245));
#11952=CARTESIAN_POINT('Ctrl Pts',(0.873158080166742,-0.0925528133349865,
0.62914037979579));
#11953=CARTESIAN_POINT('Ctrl Pts',(0.876916659919095,-0.05953,0.623857181492959));
#11954=CARTESIAN_POINT('',(0.437601487681057,-0.05953,1.03511272300331));
#11955=CARTESIAN_POINT('Origin',(0.685838782044607,-0.05953,0.860014630714833));
#11956=CARTESIAN_POINT('',(0.911784794170997,-0.05953,0.656964154625313));
#11957=CARTESIAN_POINT('Ctrl Pts',(0.911784794170998,-0.0595300000000001,
0.656964154625312));
#11958=CARTESIAN_POINT('Ctrl Pts',(0.909827729890942,-0.0762225747374255,
0.659680317203144));
#11959=CARTESIAN_POINT('Ctrl Pts',(0.907004864562642,-0.0928409665394228,
0.663576540841106));
#11960=CARTESIAN_POINT('Ctrl Pts',(0.895234408667242,-0.144299303100741,
0.679480524217551));
#11961=CARTESIAN_POINT('Ctrl Pts',(0.882797231409153,-0.177024326825049,
0.695831250979106));
#11962=CARTESIAN_POINT('Ctrl Pts',(0.854332839576145,-0.227269801620064,
0.73042219438957));
#11963=CARTESIAN_POINT('Ctrl Pts',(0.834863020612702,-0.251265615809407,
0.752807465209441));
#11964=CARTESIAN_POINT('Ctrl Pts',(0.800439809856111,-0.279889827963178,
0.789147407129766));
#11965=CARTESIAN_POINT('Ctrl Pts',(0.781998747691871,-0.290879136862659,
0.80756613568454));
#11966=CARTESIAN_POINT('Ctrl Pts',(0.742239891936898,-0.305251990234487,
0.844254137480382));
#11967=CARTESIAN_POINT('Ctrl Pts',(0.720906778729541,-0.308638795020976,
0.862505527716294));
#11968=CARTESIAN_POINT('Ctrl Pts',(0.680463863683392,-0.308638795020976,
0.894757676234429));
#11969=CARTESIAN_POINT('Ctrl Pts',(0.657923009631182,-0.305251990234488,
0.91149460735272));
#11970=CARTESIAN_POINT('Ctrl Pts',(0.613307674922609,-0.290879136862659,
0.942092777160053));
#11971=CARTESIAN_POINT('Ctrl Pts',(0.591247219971725,-0.279889827963178,
0.955972930713954));
#11972=CARTESIAN_POINT('Ctrl Pts',(0.548158511259202,-0.251265615809407,
0.981446681891443));
#11973=CARTESIAN_POINT('Ctrl Pts',(0.522002043615455,-0.227269801620063,
0.995447160474328));
#11974=CARTESIAN_POINT('Ctrl Pts',(0.481944444320713,-0.177024326825049,
1.01550068154148));
#11975=CARTESIAN_POINT('Ctrl Pts',(0.463236132117164,-0.14429930310074,
1.0239876538093));
#11976=CARTESIAN_POINT('Ctrl Pts',(0.445111721969657,-0.0928409665394226,
1.03192403056628));
#11977=CARTESIAN_POINT('Ctrl Pts',(0.440685038163619,-0.0762225747374254,
1.03380912944435));
#11978=CARTESIAN_POINT('Ctrl Pts',(0.437601487681056,-0.05953,1.03511272300331));
#11979=CARTESIAN_POINT('Origin',(0.685838782044607,-0.05953,0.860014630714833));
#11980=CARTESIAN_POINT('Origin',(0.,-0.208355,0.));
#11981=CARTESIAN_POINT('',(0.0548532617164168,-0.05953,1.12247250791415));
#11982=CARTESIAN_POINT('Origin',(0.,-0.05953,0.));
#11983=CARTESIAN_POINT('',(-0.536443649899848,-0.05953,0.987512846410683));
#11984=CARTESIAN_POINT('Ctrl Pts',(0.0548532617164173,-0.0595300000000001,
1.12247250791414));
#11985=CARTESIAN_POINT('Ctrl Pts',(0.05150947068137,-0.0762225747374254,
1.12263591311425));
#11986=CARTESIAN_POINT('Ctrl Pts',(0.0467032526342597,-0.0928409665394227,
1.12285816383385));
#11987=CARTESIAN_POINT('Ctrl Pts',(0.0269302585198975,-0.144299303100741,
1.12357162229597));
#11988=CARTESIAN_POINT('Ctrl Pts',(0.006392292392153,-0.177024326825049,
1.12404235695137));
#11989=CARTESIAN_POINT('Ctrl Pts',(-0.0383992541984087,-0.227269801620063,
1.12335509974011));
#11990=CARTESIAN_POINT('Ctrl Pts',(-0.0680399972366993,-0.251265615809407,
1.12208997038458));
#11991=CARTESIAN_POINT('Ctrl Pts',(-0.117914228755037,-0.279889827963178,
1.1178344036749));
#11992=CARTESIAN_POINT('Ctrl Pts',(-0.14381238480104,-0.290879136862659,
1.11490049012186));
#11993=CARTESIAN_POINT('Ctrl Pts',(-0.19728546073067,-0.305251990234488,
1.10669035995599));
#11994=CARTESIAN_POINT('Ctrl Pts',(-0.224855950742601,-0.308638795020976,
1.10139101611326));
#11995=CARTESIAN_POINT('Ctrl Pts',(-0.275287440920027,-0.308638795020976,
1.0898803575765));
#11996=CARTESIAN_POINT('Ctrl Pts',(-0.302426893214945,-0.305251990234488,
1.08269251410343));
#11997=CARTESIAN_POINT('Ctrl Pts',(-0.35416671187353,-0.290879136862659,
1.06688848765783));
#11998=CARTESIAN_POINT('Ctrl Pts',(-0.3787731215897,-0.279889827963178,
1.05829506364875));
#11999=CARTESIAN_POINT('Ctrl Pts',(-0.425554672694338,-0.251265615809407,
1.04048957871266));
#12000=CARTESIAN_POINT('Ctrl Pts',(-0.452808978448581,-0.227269801620063,
1.02876878445619));
#12001=CARTESIAN_POINT('Ctrl Pts',(-0.493462957200432,-0.177024326825049,
1.0099536580922));
#12002=CARTESIAN_POINT('Ctrl Pts',(-0.511762781179148,-0.14429930310074,
1.00061845128527));
#12003=CARTESIAN_POINT('Ctrl Pts',(-0.529268075276157,-0.0928409665394226,
0.991396466802468));
#12004=CARTESIAN_POINT('Ctrl Pts',(-0.533501897135713,-0.0762225747374254,
0.989110885965947));
#12005=CARTESIAN_POINT('Ctrl Pts',(-0.536443649899848,-0.0595300000000001,
0.987512846410683));
#12006=CARTESIAN_POINT('',(-0.843383895613249,-0.05953,0.742736168477219));
#12007=CARTESIAN_POINT('Origin',(0.,-0.05953,0.));
#12008=CARTESIAN_POINT('',(-1.10653577764992,-0.05953,0.196295654879792));
#12009=CARTESIAN_POINT('Ctrl Pts',(-0.843383895613249,-0.0595300000000001,
0.742736168477219));
#12010=CARTESIAN_POINT('Ctrl Pts',(-0.84559647055299,-0.0762225747374255,
0.740223768851062));
#12011=CARTESIAN_POINT('Ctrl Pts',(-0.848766861100456,-0.0928409665394227,
0.736604687327351));
#12012=CARTESIAN_POINT('Ctrl Pts',(-0.861652925570091,-0.144299303100741,
0.721590372101268));
#12013=CARTESIAN_POINT('Ctrl Pts',(-0.87482617317514,-0.177024326825049,
0.705826641853758));
#12014=CARTESIAN_POINT('Ctrl Pts',(-0.902215926359523,-0.227269801620063,
0.670378702718353));
#12015=CARTESIAN_POINT('Ctrl Pts',(-0.919707509403859,-0.251265615809407,
0.646415841396062));
#12016=CARTESIAN_POINT('Ctrl Pts',(-0.947476448101718,-0.279889827963178,
0.604769294586516));
#12017=CARTESIAN_POINT('Ctrl Pts',(-0.961329858300736,-0.290879136862659,
0.582692035672022));
#12018=CARTESIAN_POINT('Ctrl Pts',(-0.988250837578047,-0.305251990234488,
0.535766169015486));
#12019=CARTESIAN_POINT('Ctrl Pts',(-1.00129756308006,-0.308638795020976,
0.510906605094603));
#12020=CARTESIAN_POINT('Ctrl Pts',(-1.02374168767024,-0.308638795020976,
0.46430090015576));
#12021=CARTESIAN_POINT('Ctrl Pts',(-1.03504317708586,-0.305251990234488,
0.438600874831839));
#12022=CARTESIAN_POINT('Ctrl Pts',(-1.05494634094458,-0.290879136862659,
0.388295406390235));
#12023=CARTESIAN_POINT('Ctrl Pts',(-1.06356957703048,-0.279889827963178,
0.363699428370917));
#12024=CARTESIAN_POINT('Ctrl Pts',(-1.0788165083757,-0.251265615809407,
0.316022600643821));
#12025=CARTESIAN_POINT('Ctrl Pts',(-1.08664560412098,-0.227269801620063,
0.287406530683752));
#12026=CARTESIAN_POINT('Ctrl Pts',(-1.09728268713976,-0.177024326825049,
0.243890930799337));
#12027=CARTESIAN_POINT('Ctrl Pts',(-1.10139388218929,-0.144299303100741,
0.22376314604679));
#12028=CARTESIAN_POINT('Ctrl Pts',(-1.10509821673782,-0.0928409665394227,
0.204327142733961));
#12029=CARTESIAN_POINT('Ctrl Pts',(-1.10595102243643,-0.0762225747374254,
0.199591971170104));
#12030=CARTESIAN_POINT('Ctrl Pts',(-1.10653577764992,-0.0595300000000001,
0.196295654879792));
#12031=CARTESIAN_POINT('',(-1.123812,-0.05953,1.37627276864339E-16));
#12032=CARTESIAN_POINT('Origin',(0.,-0.05953,0.));
#12033=CARTESIAN_POINT('',(-1.123812,-0.35718,1.37627276864339E-16));
#12034=CARTESIAN_POINT('',(-1.123812,-0.208355,1.37627276864339E-16));
#12035=CARTESIAN_POINT('Origin',(0.,-0.35718,0.));
#12036=CARTESIAN_POINT('',(-1.10653577764992,-0.05953,-0.196295654879793));
#12037=CARTESIAN_POINT('Origin',(0.,-0.05953,0.));
#12038=CARTESIAN_POINT('',(-0.843383895613249,-0.05953,-0.742736168477219));
#12039=CARTESIAN_POINT('Ctrl Pts',(-1.10653577764992,-0.0595300000000001,
-0.196295654879792));
#12040=CARTESIAN_POINT('Ctrl Pts',(-1.10595102243643,-0.0762225747374255,
-0.199591971170104));
#12041=CARTESIAN_POINT('Ctrl Pts',(-1.10509821673782,-0.0928409665394228,
-0.204327142733962));
#12042=CARTESIAN_POINT('Ctrl Pts',(-1.10139388218929,-0.144299303100741,
-0.22376314604679));
#12043=CARTESIAN_POINT('Ctrl Pts',(-1.09728268713976,-0.177024326825049,
-0.243890930799338));
#12044=CARTESIAN_POINT('Ctrl Pts',(-1.08664560412098,-0.227269801620063,
-0.287406530683753));
#12045=CARTESIAN_POINT('Ctrl Pts',(-1.0788165083757,-0.251265615809407,
-0.316022600643821));
#12046=CARTESIAN_POINT('Ctrl Pts',(-1.06356957703048,-0.279889827963178,
-0.363699428370918));
#12047=CARTESIAN_POINT('Ctrl Pts',(-1.05494634094458,-0.290879136862659,
-0.388295406390235));
#12048=CARTESIAN_POINT('Ctrl Pts',(-1.03504317708586,-0.305251990234488,
-0.438600874831839));
#12049=CARTESIAN_POINT('Ctrl Pts',(-1.02374168767024,-0.308638795020976,
-0.46430090015576));
#12050=CARTESIAN_POINT('Ctrl Pts',(-1.00129756308006,-0.308638795020976,
-0.510906605094603));
#12051=CARTESIAN_POINT('Ctrl Pts',(-0.988250837578047,-0.305251990234488,
-0.535766169015486));
#12052=CARTESIAN_POINT('Ctrl Pts',(-0.961329858300736,-0.290879136862659,
-0.582692035672022));
#12053=CARTESIAN_POINT('Ctrl Pts',(-0.947476448101718,-0.279889827963178,
-0.604769294586516));
#12054=CARTESIAN_POINT('Ctrl Pts',(-0.919707509403859,-0.251265615809407,
-0.646415841396062));
#12055=CARTESIAN_POINT('Ctrl Pts',(-0.902215926359523,-0.227269801620064,
-0.670378702718353));
#12056=CARTESIAN_POINT('Ctrl Pts',(-0.87482617317514,-0.177024326825049,
-0.705826641853758));
#12057=CARTESIAN_POINT('Ctrl Pts',(-0.861652925570091,-0.144299303100741,
-0.721590372101268));
#12058=CARTESIAN_POINT('Ctrl Pts',(-0.848766861100456,-0.0928409665394229,
-0.736604687327351));
#12059=CARTESIAN_POINT('Ctrl Pts',(-0.84559647055299,-0.0762225747374255,
-0.740223768851063));
#12060=CARTESIAN_POINT('Ctrl Pts',(-0.843383895613249,-0.0595300000000001,
-0.742736168477219));
#12061=CARTESIAN_POINT('',(-0.536443649899847,-0.05953,-0.987512846410683));
#12062=CARTESIAN_POINT('Origin',(0.,-0.05953,0.));
#12063=CARTESIAN_POINT('',(0.0548532617164172,-0.05953,-1.12247250791415));
#12064=CARTESIAN_POINT('Ctrl Pts',(-0.536443649899848,-0.0595300000000001,
-0.987512846410683));
#12065=CARTESIAN_POINT('Ctrl Pts',(-0.533501897135712,-0.0762225747374254,
-0.989110885965947));
#12066=CARTESIAN_POINT('Ctrl Pts',(-0.529268075276156,-0.0928409665394227,
-0.991396466802469));
#12067=CARTESIAN_POINT('Ctrl Pts',(-0.511762781179147,-0.144299303100741,
-1.00061845128527));
#12068=CARTESIAN_POINT('Ctrl Pts',(-0.493462957200432,-0.177024326825049,
-1.0099536580922));
#12069=CARTESIAN_POINT('Ctrl Pts',(-0.45280897844858,-0.227269801620063,
-1.02876878445619));
#12070=CARTESIAN_POINT('Ctrl Pts',(-0.425554672694337,-0.251265615809407,
-1.04048957871266));
#12071=CARTESIAN_POINT('Ctrl Pts',(-0.3787731215897,-0.279889827963178,
-1.05829506364875));
#12072=CARTESIAN_POINT('Ctrl Pts',(-0.354166711873529,-0.290879136862659,
-1.06688848765783));
#12073=CARTESIAN_POINT('Ctrl Pts',(-0.302426893214944,-0.305251990234488,
-1.08269251410343));
#12074=CARTESIAN_POINT('Ctrl Pts',(-0.275287440920027,-0.308638795020976,
-1.0898803575765));
#12075=CARTESIAN_POINT('Ctrl Pts',(-0.224855950742601,-0.308638795020976,
-1.10139101611326));
#12076=CARTESIAN_POINT('Ctrl Pts',(-0.19728546073067,-0.305251990234488,
-1.10669035995599));
#12077=CARTESIAN_POINT('Ctrl Pts',(-0.143812384801039,-0.290879136862659,
-1.11490049012186));
#12078=CARTESIAN_POINT('Ctrl Pts',(-0.117914228755037,-0.279889827963178,
-1.1178344036749));
#12079=CARTESIAN_POINT('Ctrl Pts',(-0.0680399972366989,-0.251265615809407,
-1.12208997038458));
#12080=CARTESIAN_POINT('Ctrl Pts',(-0.0383992541984084,-0.227269801620063,
-1.12335509974011));
#12081=CARTESIAN_POINT('Ctrl Pts',(0.00639229239215326,-0.177024326825049,
-1.12404235695137));
#12082=CARTESIAN_POINT('Ctrl Pts',(0.0269302585198977,-0.144299303100741,
-1.12357162229597));
#12083=CARTESIAN_POINT('Ctrl Pts',(0.04670325263426,-0.0928409665394228,
-1.12285816383385));
#12084=CARTESIAN_POINT('Ctrl Pts',(0.0515094706813703,-0.0762225747374255,
-1.12263591311425));
#12085=CARTESIAN_POINT('Ctrl Pts',(0.0548532617164176,-0.0595300000000001,
-1.12247250791414));
#12086=CARTESIAN_POINT('',(0.437601487681057,-0.05953,-1.03511272300331));
#12087=CARTESIAN_POINT('Origin',(0.,-0.05953,0.));
#12088=CARTESIAN_POINT('',(0.911784794170997,-0.05953,-0.656964154625313));
#12089=CARTESIAN_POINT('Ctrl Pts',(0.437601487681056,-0.0595300000000001,
-1.03511272300331));
#12090=CARTESIAN_POINT('Ctrl Pts',(0.440685038163619,-0.0762225747374255,
-1.03380912944435));
#12091=CARTESIAN_POINT('Ctrl Pts',(0.445111721969657,-0.0928409665394228,
-1.03192403056628));
#12092=CARTESIAN_POINT('Ctrl Pts',(0.463236132117164,-0.144299303100741,
-1.0239876538093));
#12093=CARTESIAN_POINT('Ctrl Pts',(0.481944444320713,-0.177024326825049,
-1.01550068154148));
#12094=CARTESIAN_POINT('Ctrl Pts',(0.522002043615455,-0.227269801620064,
-0.995447160474328));
#12095=CARTESIAN_POINT('Ctrl Pts',(0.548158511259203,-0.251265615809407,
-0.981446681891443));
#12096=CARTESIAN_POINT('Ctrl Pts',(0.591247219971725,-0.279889827963178,
-0.955972930713954));
#12097=CARTESIAN_POINT('Ctrl Pts',(0.613307674922609,-0.290879136862659,
-0.942092777160053));
#12098=CARTESIAN_POINT('Ctrl Pts',(0.657923009631182,-0.305251990234487,
-0.91149460735272));
#12099=CARTESIAN_POINT('Ctrl Pts',(0.680463863683393,-0.308638795020976,
-0.894757676234429));
#12100=CARTESIAN_POINT('Ctrl Pts',(0.720906778729542,-0.308638795020976,
-0.862505527716294));
#12101=CARTESIAN_POINT('Ctrl Pts',(0.742239891936899,-0.305251990234488,
-0.844254137480381));
#12102=CARTESIAN_POINT('Ctrl Pts',(0.781998747691872,-0.290879136862659,
-0.80756613568454));
#12103=CARTESIAN_POINT('Ctrl Pts',(0.800439809856112,-0.279889827963178,
-0.789147407129765));
#12104=CARTESIAN_POINT('Ctrl Pts',(0.834863020612702,-0.251265615809407,
-0.752807465209441));
#12105=CARTESIAN_POINT('Ctrl Pts',(0.854332839576145,-0.227269801620064,
-0.73042219438957));
#12106=CARTESIAN_POINT('Ctrl Pts',(0.882797231409153,-0.177024326825049,
-0.695831250979106));
#12107=CARTESIAN_POINT('Ctrl Pts',(0.895234408667242,-0.144299303100741,
-0.679480524217551));
#12108=CARTESIAN_POINT('Ctrl Pts',(0.907004864562642,-0.0928409665394228,
-0.663576540841106));
#12109=CARTESIAN_POINT('Ctrl Pts',(0.909827729890942,-0.0762225747374256,
-0.659680317203144));
#12110=CARTESIAN_POINT('Ctrl Pts',(0.911784794170998,-0.0595300000000001,
-0.656964154625312));
#12111=CARTESIAN_POINT('',(1.08212377959455,-0.05953,-0.303251606722892));
#12112=CARTESIAN_POINT('Origin',(0.,-0.05953,0.));
#12113=CARTESIAN_POINT('',(1.08212377959455,-0.05953,0.303251606722892));
#12114=CARTESIAN_POINT('Ctrl Pts',(1.08212377959455,-0.0595300000000001,
-0.303251606722892));
#12115=CARTESIAN_POINT('Ctrl Pts',(1.0830271513892,-0.0762225747374255,
-0.300028012588062));
#12116=CARTESIAN_POINT('Ctrl Pts',(1.08431331394788,-0.0928409665394228,
-0.2953917518996));
#12117=CARTESIAN_POINT('Ctrl Pts',(1.08940878963422,-0.144299303100741,
-0.276273267473431));
#12118=CARTESIAN_POINT('Ctrl Pts',(1.09443784939331,-0.177024326825049,
-0.256354979351213));
#12119=CARTESIAN_POINT('Ctrl Pts',(1.10373487993589,-0.227269801620064,
-0.212533521233765));
#12120=CARTESIAN_POINT('Ctrl Pts',(1.10909715583869,-0.251265615809407,
-0.183354415742157));
#12121=CARTESIAN_POINT('Ctrl Pts',(1.1160463456491,-0.279889827963178,-0.133783682657561));
#12122=CARTESIAN_POINT('Ctrl Pts',(1.11894887330541,-0.290879136862659,
-0.107881990270302));
#12123=CARTESIAN_POINT('Ctrl Pts',(1.12284346704144,-0.305251990234488,
-0.0539226701638766));
#12124=CARTESIAN_POINT('Ctrl Pts',(1.123812,-0.308638795020976,-0.025864214957475));
#12125=CARTESIAN_POINT('Ctrl Pts',(1.123812,-0.308638795020976,0.025864214957475));
#12126=CARTESIAN_POINT('Ctrl Pts',(1.12284346704144,-0.305251990234488,
0.0539226701638766));
#12127=CARTESIAN_POINT('Ctrl Pts',(1.11894887330541,-0.290879136862659,
0.107881990270302));
#12128=CARTESIAN_POINT('Ctrl Pts',(1.1160463456491,-0.279889827963178,0.133783682657561));
#12129=CARTESIAN_POINT('Ctrl Pts',(1.10909715583869,-0.251265615809407,
0.183354415742157));
#12130=CARTESIAN_POINT('Ctrl Pts',(1.10373487993589,-0.227269801620064,
0.212533521233765));
#12131=CARTESIAN_POINT('Ctrl Pts',(1.09443784939331,-0.177024326825049,
0.256354979351213));
#12132=CARTESIAN_POINT('Ctrl Pts',(1.08940878963422,-0.144299303100741,
0.276273267473431));
#12133=CARTESIAN_POINT('Ctrl Pts',(1.08431331394788,-0.0928409665394228,
0.2953917518996));
#12134=CARTESIAN_POINT('Ctrl Pts',(1.0830271513892,-0.0762225747374255,
0.300028012588062));
#12135=CARTESIAN_POINT('Ctrl Pts',(1.08212377959455,-0.0595300000000001,
0.303251606722892));
#12136=CARTESIAN_POINT('Origin',(0.,-0.05953,0.));
#12137=CARTESIAN_POINT('Origin',(0.,-0.05953,0.));
#12138=CARTESIAN_POINT('',(0.0589974094846122,-0.05953,1.07456964270265));
#12139=CARTESIAN_POINT('Origin',(0.,-0.05953,0.));
#12140=CARTESIAN_POINT('Origin',(-0.244773027351946,-0.05953,1.07242070340001));
#12141=CARTESIAN_POINT('Origin',(-0.244773027351946,0.,1.07242070340001));
#12142=CARTESIAN_POINT('',(-0.519393123750572,-0.05953,0.942555777842682));
#12143=CARTESIAN_POINT('Ctrl Pts',(-0.519393123750572,-0.05953,0.942555777842682));
#12144=CARTESIAN_POINT('Ctrl Pts',(-0.513714466572041,-0.0925528133349865,
0.945684988399766));
#12145=CARTESIAN_POINT('Ctrl Pts',(-0.503136848051455,-0.124911173756694,
0.951483858396181));
#12146=CARTESIAN_POINT('Ctrl Pts',(-0.47593627990192,-0.177924977804098,
0.965323333309091));
#12147=CARTESIAN_POINT('Ctrl Pts',(-0.460931856495794,-0.199697230012983,
0.972669835243841));
#12148=CARTESIAN_POINT('Ctrl Pts',(-0.426157505475872,-0.237895043532788,
0.988400002689705));
#12149=CARTESIAN_POINT('Ctrl Pts',(-0.406380688682952,-0.254319232363049,
0.996771768218699));
#12150=CARTESIAN_POINT('Ctrl Pts',(-0.364750145543744,-0.28018331644634,
1.01272583306292));
#12151=CARTESIAN_POINT('Ctrl Pts',(-0.340838910881557,-0.29104845371857,
1.02112815447116));
#12152=CARTESIAN_POINT('Ctrl Pts',(-0.290495481564827,-0.30527573347708,
1.036574285215));
#12153=CARTESIAN_POINT('Ctrl Pts',(-0.264056468041074,-0.308638795020976,
1.04359501395068));
#12154=CARTESIAN_POINT('Ctrl Pts',(-0.214892249704082,-0.308638795020976,
1.05481642595959));
#12155=CARTESIAN_POINT('Ctrl Pts',(-0.188025341585962,-0.30527573347708,
1.05996242598502));
#12156=CARTESIAN_POINT('Ctrl Pts',(-0.135965654106109,-0.29104845371857,
1.06788913840721));
#12157=CARTESIAN_POINT('Ctrl Pts',(-0.110776745452494,-0.28018331644634,
1.07069360430242));
#12158=CARTESIAN_POINT('Ctrl Pts',(-0.0663467128214646,-0.254319232363049,
1.07438230428002));
#12159=CARTESIAN_POINT('Ctrl Pts',(-0.0448960436540983,-0.237895043532788,
1.07542044338697));
#12160=CARTESIAN_POINT('Ctrl Pts',(-0.00674037211528124,-0.199697230012983,
1.07633607767727));
#12161=CARTESIAN_POINT('Ctrl Pts',(0.00996567398334777,-0.177924977804098,
1.07622728347683));
#12162=CARTESIAN_POINT('Ctrl Pts',(0.0404772621979741,-0.124911173756694,
1.07556023164702));
#12163=CARTESIAN_POINT('Ctrl Pts',(0.0525234025782719,-0.0925528133349865,
1.07492508698591));
#12164=CARTESIAN_POINT('Ctrl Pts',(0.0589974094846124,-0.05953,1.07456964270265));
#12165=CARTESIAN_POINT('Origin',(-0.244773027351946,-0.05953,1.07242070340001));
#12166=CARTESIAN_POINT('Origin',(0.,-0.05953,0.));
#12167=CARTESIAN_POINT('',(-0.803348093619616,-0.05953,0.716109245731214));
#12168=CARTESIAN_POINT('Origin',(0.,-0.05953,0.));
#12169=CARTESIAN_POINT('Origin',(-0.991065754692661,-0.05953,0.477272113029314));
#12170=CARTESIAN_POINT('Origin',(-0.991065754692661,0.,0.477272113029314));
#12171=CARTESIAN_POINT('',(-1.06075609691358,-0.05953,0.181596019242328));
#12172=CARTESIAN_POINT('Ctrl Pts',(-1.06075609691358,-0.05953,0.181596019242328));
#12173=CARTESIAN_POINT('Ctrl Pts',(-1.05966202740332,-0.0925528133349865,
0.187986803072856));
#12174=CARTESIAN_POINT('Ctrl Pts',(-1.05760072925372,-0.124911173756694,
0.199872254546857));
#12175=CARTESIAN_POINT('Ctrl Pts',(-1.05146158959546,-0.177924977804098,
0.22976728653846));
#12176=CARTESIAN_POINT('Ctrl Pts',(-1.04785021111757,-0.199697230012983,
0.246078686169301));
#12177=CARTESIAN_POINT('Ctrl Pts',(-1.03846709802406,-0.237895043532788,
0.283073967563097));
#12178=CARTESIAN_POINT('Ctrl Pts',(-1.03268176429485,-0.254319232363049,
0.303755815985685));
#12179=CARTESIAN_POINT('Ctrl Pts',(-1.01919893537026,-0.28018331644634,
0.346251081972725));
#12180=CARTESIAN_POINT('Ctrl Pts',(-1.01085972381132,-0.29104845371857,
0.370184399726282));
#12181=CARTESIAN_POINT('Ctrl Pts',(-0.99154738033959,-0.30527573347708,
0.419174982698463));
#12182=CARTESIAN_POINT('Ctrl Pts',(-0.980551951791748,-0.308638795020976,
0.444223188605045));
#12183=CARTESIAN_POINT('Ctrl Pts',(-0.958671816228589,-0.308638795020976,
0.489657758261848));
#12184=CARTESIAN_POINT('Ctrl Pts',(-0.945943877838127,-0.30527573347708,
0.51387163140139));
#12185=CARTESIAN_POINT('Ctrl Pts',(-0.91968254693063,-0.29104845371857,
0.559515758398093));
#12186=CARTESIAN_POINT('Ctrl Pts',(-0.906170138993533,-0.28018331644634,
0.580957796077825));
#12187=CARTESIAN_POINT('Ctrl Pts',(-0.8813524085237,-0.254319232363049,
0.617994461173994));
#12188=CARTESIAN_POINT('Ctrl Pts',(-0.868789784891799,-0.237895043532788,
0.635412538795143));
#12189=CARTESIAN_POINT('Ctrl Pts',(-0.845715984518854,-0.199697230012983,
0.66581473268113));
#12190=CARTESIAN_POINT('Ctrl Pts',(-0.835214876415962,-0.177924977804098,
0.678808213394124));
#12191=CARTESIAN_POINT('Ctrl Pts',(-0.815669690204649,-0.124911173756694,
0.702247233627224));
#12192=CARTESIAN_POINT('Ctrl Pts',(-0.807662468433796,-0.0925528133349865,
0.711269279199861));
#12193=CARTESIAN_POINT('Ctrl Pts',(-0.803348093619616,-0.05953,0.716109245731214));
#12194=CARTESIAN_POINT('Origin',(-0.991065754692661,-0.05953,0.477272113029314));
#12195=CARTESIAN_POINT('Origin',(0.,-0.05953,0.));
#12196=CARTESIAN_POINT('',(-1.076188,-0.05953,1.31795018948079E-16));
#12197=CARTESIAN_POINT('Origin',(0.,-0.05953,0.));
#12198=CARTESIAN_POINT('',(-1.06075609691358,-0.05953,-0.181596019242328));
#12199=CARTESIAN_POINT('Origin',(0.,-0.05953,0.));
#12200=CARTESIAN_POINT('Origin',(-0.991065754692661,-0.05953,-0.477272113029314));
#12201=CARTESIAN_POINT('Origin',(-0.991065754692661,0.,-0.477272113029314));
#12202=CARTESIAN_POINT('',(-0.803348093619616,-0.05953,-0.716109245731215));
#12203=CARTESIAN_POINT('Ctrl Pts',(-0.803348093619616,-0.05953,-0.716109245731215));
#12204=CARTESIAN_POINT('Ctrl Pts',(-0.807662468433795,-0.0925528133349865,
-0.711269279199862));
#12205=CARTESIAN_POINT('Ctrl Pts',(-0.815669690204649,-0.124911173756694,
-0.702247233627224));
#12206=CARTESIAN_POINT('Ctrl Pts',(-0.835214876415962,-0.177924977804098,
-0.678808213394124));
#12207=CARTESIAN_POINT('Ctrl Pts',(-0.845715984518854,-0.199697230012983,
-0.66581473268113));
#12208=CARTESIAN_POINT('Ctrl Pts',(-0.868789784891799,-0.237895043532788,
-0.635412538795143));
#12209=CARTESIAN_POINT('Ctrl Pts',(-0.8813524085237,-0.254319232363049,
-0.617994461173994));
#12210=CARTESIAN_POINT('Ctrl Pts',(-0.906170138993533,-0.28018331644634,
-0.580957796077826));
#12211=CARTESIAN_POINT('Ctrl Pts',(-0.91968254693063,-0.29104845371857,
-0.559515758398093));
#12212=CARTESIAN_POINT('Ctrl Pts',(-0.945943877838127,-0.30527573347708,
-0.51387163140139));
#12213=CARTESIAN_POINT('Ctrl Pts',(-0.958671816228589,-0.308638795020976,
-0.489657758261848));
#12214=CARTESIAN_POINT('Ctrl Pts',(-0.980551951791748,-0.308638795020976,
-0.444223188605045));
#12215=CARTESIAN_POINT('Ctrl Pts',(-0.99154738033959,-0.30527573347708,
-0.419174982698463));
#12216=CARTESIAN_POINT('Ctrl Pts',(-1.01085972381132,-0.29104845371857,
-0.370184399726282));
#12217=CARTESIAN_POINT('Ctrl Pts',(-1.01919893537026,-0.28018331644634,
-0.346251081972725));
#12218=CARTESIAN_POINT('Ctrl Pts',(-1.03268176429485,-0.254319232363049,
-0.303755815985685));
#12219=CARTESIAN_POINT('Ctrl Pts',(-1.03846709802406,-0.237895043532788,
-0.283073967563097));
#12220=CARTESIAN_POINT('Ctrl Pts',(-1.04785021111757,-0.199697230012983,
-0.246078686169302));
#12221=CARTESIAN_POINT('Ctrl Pts',(-1.05146158959546,-0.177924977804098,
-0.229767286538461));
#12222=CARTESIAN_POINT('Ctrl Pts',(-1.05760072925372,-0.124911173756694,
-0.199872254546858));
#12223=CARTESIAN_POINT('Ctrl Pts',(-1.05966202740332,-0.0925528133349864,
-0.187986803072857));
#12224=CARTESIAN_POINT('Ctrl Pts',(-1.06075609691358,-0.05953,-0.181596019242328));
#12225=CARTESIAN_POINT('Origin',(-0.991065754692661,-0.05953,-0.477272113029314));
#12226=CARTESIAN_POINT('Origin',(0.,-0.05953,0.));
#12227=CARTESIAN_POINT('',(-0.519393123750572,-0.05953,-0.942555777842682));
#12228=CARTESIAN_POINT('Origin',(0.,-0.05953,0.));
#12229=CARTESIAN_POINT('Origin',(-0.244773027351946,-0.05953,-1.07242070340001));
#12230=CARTESIAN_POINT('Origin',(-0.244773027351946,0.,-1.07242070340001));
#12231=CARTESIAN_POINT('',(0.0589974094846125,-0.05953,-1.07456964270265));
#12232=CARTESIAN_POINT('Ctrl Pts',(0.0589974094846127,-0.05953,-1.07456964270265));
#12233=CARTESIAN_POINT('Ctrl Pts',(0.0525234025782722,-0.0925528133349865,
-1.07492508698591));
#12234=CARTESIAN_POINT('Ctrl Pts',(0.0404772621979744,-0.124911173756694,
-1.07556023164702));
#12235=CARTESIAN_POINT('Ctrl Pts',(0.0099656739833481,-0.177924977804098,
-1.07622728347683));
#12236=CARTESIAN_POINT('Ctrl Pts',(-0.00674037211528096,-0.199697230012983,
-1.07633607767727));
#12237=CARTESIAN_POINT('Ctrl Pts',(-0.044896043654098,-0.237895043532788,
-1.07542044338697));
#12238=CARTESIAN_POINT('Ctrl Pts',(-0.0663467128214644,-0.254319232363049,
-1.07438230428002));
#12239=CARTESIAN_POINT('Ctrl Pts',(-0.110776745452493,-0.28018331644634,
-1.07069360430242));
#12240=CARTESIAN_POINT('Ctrl Pts',(-0.135965654106109,-0.29104845371857,
-1.06788913840721));
#12241=CARTESIAN_POINT('Ctrl Pts',(-0.188025341585962,-0.30527573347708,
-1.05996242598502));
#12242=CARTESIAN_POINT('Ctrl Pts',(-0.214892249704082,-0.308638795020976,
-1.05481642595959));
#12243=CARTESIAN_POINT('Ctrl Pts',(-0.264056468041074,-0.308638795020976,
-1.04359501395068));
#12244=CARTESIAN_POINT('Ctrl Pts',(-0.290495481564827,-0.30527573347708,
-1.036574285215));
#12245=CARTESIAN_POINT('Ctrl Pts',(-0.340838910881557,-0.291048453718569,
-1.02112815447116));
#12246=CARTESIAN_POINT('Ctrl Pts',(-0.364750145543744,-0.28018331644634,
-1.01272583306292));
#12247=CARTESIAN_POINT('Ctrl Pts',(-0.406380688682952,-0.254319232363049,
-0.996771768218699));
#12248=CARTESIAN_POINT('Ctrl Pts',(-0.426157505475872,-0.237895043532788,
-0.988400002689705));
#12249=CARTESIAN_POINT('Ctrl Pts',(-0.460931856495794,-0.199697230012983,
-0.972669835243841));
#12250=CARTESIAN_POINT('Ctrl Pts',(-0.475936279901919,-0.177924977804098,
-0.965323333309091));
#12251=CARTESIAN_POINT('Ctrl Pts',(-0.503136848051454,-0.124911173756694,
-0.951483858396181));
#12252=CARTESIAN_POINT('Ctrl Pts',(-0.513714466572041,-0.0925528133349865,
-0.945684988399766));
#12253=CARTESIAN_POINT('Ctrl Pts',(-0.519393123750572,-0.05953,-0.942555777842682));
#12254=CARTESIAN_POINT('Origin',(-0.244773027351946,-0.05953,-1.07242070340001));
#12255=CARTESIAN_POINT('Origin',(0.,-0.05953,0.));
#12256=CARTESIAN_POINT('',(0.413083465285518,-0.05953,-0.993751811093549));
#12257=CARTESIAN_POINT('Origin',(0.,-0.05953,0.));
#12258=CARTESIAN_POINT('Origin',(0.685838782044607,-0.05953,-0.860014630714833));
#12259=CARTESIAN_POINT('Origin',(0.685838782044607,0.,-0.860014630714833));
#12260=CARTESIAN_POINT('',(0.876916659919095,-0.05953,-0.623857181492959));
#12261=CARTESIAN_POINT('Ctrl Pts',(0.876916659919095,-0.05953,-0.623857181492958));
#12262=CARTESIAN_POINT('Ctrl Pts',(0.873158080166742,-0.0925528133349865,
-0.62914037979579));
#12263=CARTESIAN_POINT('Ctrl Pts',(0.866144010579847,-0.124911173756694,
-0.638954437806245));
#12264=CARTESIAN_POINT('Ctrl Pts',(0.847641868610495,-0.177924977804098,
-0.663225258065736));
#12265=CARTESIAN_POINT('Ctrl Pts',(0.837310877969633,-0.199697230012983,
-0.676354402927683));
#12266=CARTESIAN_POINT('Ctrl Pts',(0.81280533416753,-0.237895043532788,
-0.705614819529209));
#12267=CARTESIAN_POINT('Ctrl Pts',(0.798619410861634,-0.254319232363049,
-0.721738358858166));
#12268=CARTESIAN_POINT('Ctrl Pts',(0.768033796848072,-0.28018331644634,
-0.754175290318038));
#12269=CARTESIAN_POINT('Ctrl Pts',(0.750136149454208,-0.29104845371857,
-0.772120216227122));
#12270=CARTESIAN_POINT('Ctrl Pts',(0.711480111898423,-0.30527573347708,
-0.807879894508811));
#12271=CARTESIAN_POINT('Ctrl Pts',(0.690705563850638,-0.308638795020976,
-0.825676810575913));
#12272=CARTESIAN_POINT('Ctrl Pts',(0.651278921914856,-0.308638795020976,
-0.857118508332695));
#12273=CARTESIAN_POINT('Ctrl Pts',(0.629305439856167,-0.30527573347708,
-0.873412008702649));
#12274=CARTESIAN_POINT('Ctrl Pts',(0.585840553788742,-0.29104845371857,
-0.903141581680914));
#12275=CARTESIAN_POINT('Ctrl Pts',(0.564362943424239,-0.28018331644634,
-0.916597376014514));
#12276=CARTESIAN_POINT('Ctrl Pts',(0.525933334162556,-0.254319232363049,
-0.939198248544427));
#12277=CARTESIAN_POINT('Ctrl Pts',(0.507057380724533,-0.237895043532788,
-0.949440676105255));
#12278=CARTESIAN_POINT('Ctrl Pts',(0.473077587363686,-0.199697230012983,
-0.966820759530997));
#12279=CARTESIAN_POINT('Ctrl Pts',(0.457978755888596,-0.177924977804098,
-0.973971221090534));
#12280=CARTESIAN_POINT('Ctrl Pts',(0.430199341854858,-0.124911173756694,
-0.986608710139579));
#12281=CARTESIAN_POINT('Ctrl Pts',(0.419070565453384,-0.0925528133349865,
-0.991263089003441));
#12282=CARTESIAN_POINT('Ctrl Pts',(0.413083465285518,-0.05953,-0.993751811093549));
#12283=CARTESIAN_POINT('Origin',(0.685838782044607,-0.05953,-0.860014630714833));
#12284=CARTESIAN_POINT('Origin',(0.,-0.208355,0.));
#12285=CARTESIAN_POINT('',(-1.076188,-0.35718,1.31795018948079E-16));
#12286=CARTESIAN_POINT('Origin',(0.,-0.35718,0.));
#12287=CARTESIAN_POINT('',(-1.076188,-0.208355,1.31795018948079E-16));
#12288=CARTESIAN_POINT('',(1.03449977959455,-0.05953,0.296632461748266));
#12289=CARTESIAN_POINT('Origin',(0.,-0.05953,0.));
#12290=CARTESIAN_POINT('',(1.03449977959455,-0.05953,-0.296632461748266));
#12291=CARTESIAN_POINT('Ctrl Pts',(1.03449977959455,-0.05953,0.296632461748267));
#12292=CARTESIAN_POINT('Ctrl Pts',(1.03628691421076,-0.0925528133349865,
0.290399865505497));
#12293=CARTESIAN_POINT('Ctrl Pts',(1.03958665287714,-0.124911173756694,
0.278797079997872));
#12294=CARTESIAN_POINT('Ctrl Pts',(1.0470264474309,-0.177924977804098,0.249198913998601));
#12295=CARTESIAN_POINT('Ctrl Pts',(1.05084995891418,-0.199697230012983,
0.232935932341942));
#12296=CARTESIAN_POINT('Ctrl Pts',(1.05844771715377,-0.237895043532788,
0.195533155353269));
#12297=CARTESIAN_POINT('Ctrl Pts',(1.06220882929878,-0.254319232363049,
0.17438929156337));
#12298=CARTESIAN_POINT('Ctrl Pts',(1.06849922508772,-0.28018331644634,0.130252399648131));
#12299=CARTESIAN_POINT('Ctrl Pts',(1.07137013248666,-0.29104845371857,0.105070977154072));
#12300=CARTESIAN_POINT('Ctrl Pts',(1.07522652957392,-0.30527573347708,0.0525526752791107));
#12301=CARTESIAN_POINT('Ctrl Pts',(1.076188,-0.308638795020976,0.025214283908933));
#12302=CARTESIAN_POINT('Ctrl Pts',(1.076188,-0.308638795020976,-0.025214283908933));
#12303=CARTESIAN_POINT('Ctrl Pts',(1.07522652957392,-0.30527573347708,-0.0525526752791107));
#12304=CARTESIAN_POINT('Ctrl Pts',(1.07137013248666,-0.29104845371857,-0.105070977154072));
#12305=CARTESIAN_POINT('Ctrl Pts',(1.06849922508772,-0.28018331644634,-0.130252399648131));
#12306=CARTESIAN_POINT('Ctrl Pts',(1.06220882929878,-0.254319232363049,
-0.17438929156337));
#12307=CARTESIAN_POINT('Ctrl Pts',(1.05844771715377,-0.237895043532788,
-0.195533155353269));
#12308=CARTESIAN_POINT('Ctrl Pts',(1.05084995891418,-0.199697230012983,
-0.232935932341942));
#12309=CARTESIAN_POINT('Ctrl Pts',(1.0470264474309,-0.177924977804098,-0.249198913998601));
#12310=CARTESIAN_POINT('Ctrl Pts',(1.03958665287714,-0.124911173756694,
-0.278797079997872));
#12311=CARTESIAN_POINT('Ctrl Pts',(1.03628691421076,-0.0925528133349865,
-0.290399865505497));
#12312=CARTESIAN_POINT('Ctrl Pts',(1.03449977959455,-0.05953,-0.296632461748267));
#12313=CARTESIAN_POINT('Origin',(0.,-0.05953,0.));
#12314=CARTESIAN_POINT('Origin',(0.,-0.05953,0.));
#12315=CARTESIAN_POINT('Origin',(1.1,-0.05953,0.));
#12316=CARTESIAN_POINT('Origin',(1.1,0.,0.));
#12317=CARTESIAN_POINT('Origin',(1.1,-0.05953,0.));
#12318=CARTESIAN_POINT('Origin',(0.,-0.35718,0.));
#12319=CARTESIAN_POINT('Origin',(0.,-0.05953,0.));
#13209=UNCERTAINTY_MEASURE_WITH_UNIT(LENGTH_MEASURE(0.001),#13278,
'DISTANCE_ACCURACY_VALUE',
'Maximum model space distance between geometric entities at asserted c
onnectivities');
#13233=UNCERTAINTY_MEASURE_WITH_UNIT(LENGTH_MEASURE(0.001),#13278,
'DISTANCE_ACCURACY_VALUE',
'Maximum model space distance between geometric entities at asserted c
onnectivities');
#13253=(
GEOMETRIC_REPRESENTATION_CONTEXT(3)
GLOBAL_UNCERTAINTY_ASSIGNED_CONTEXT((#13209))
GLOBAL_UNIT_ASSIGNED_CONTEXT((#13278,#13280,#13281))
REPRESENTATION_CONTEXT('','3D')
);
#13277=(
GEOMETRIC_REPRESENTATION_CONTEXT(3)
GLOBAL_UNCERTAINTY_ASSIGNED_CONTEXT((#13233))
GLOBAL_UNIT_ASSIGNED_CONTEXT((#13278,#13280,#13281))
REPRESENTATION_CONTEXT('','3D')
);
#13278=(
LENGTH_UNIT()
NAMED_UNIT(*)
SI_UNIT(.CENTI.,.METRE.)
);
#13280=(
NAMED_UNIT(*)
PLANE_ANGLE_UNIT()
SI_UNIT($,.RADIAN.)
);
#13281=(
NAMED_UNIT(*)
SI_UNIT($,.STERADIAN.)
SOLID_ANGLE_UNIT()
);
#13301=SHAPE_DEFINITION_REPRESENTATION(#13344,#13458);
#13344=PRODUCT_DEFINITION_SHAPE('',$,#13502);
#13458=SHAPE_REPRESENTATION('',(#7210),#13253);
#13482=PRODUCT_DEFINITION_CONTEXT('part definition',#13613,'design');
#13502=PRODUCT_DEFINITION('Cage','Cage',#13545,#13482);
#13545=PRODUCT_DEFINITION_FORMATION('',$,#13634);
#13613=APPLICATION_CONTEXT(
'Core Data for Automotive Mechanical Design Process');
#13614=PRODUCT_CONTEXT('part definition',#13613,'mechanical');
#13634=PRODUCT('Cage','Cage','Cage',(#13614));
#13714=COLOUR_RGB('Grey',0.48,0.52,0.57);
#13715=FILL_AREA_STYLE_COLOUR('',#13714);
#13716=FILL_AREA_STYLE('',(#13715));
#13717=SURFACE_STYLE_FILL_AREA(#13716);
#13718=SURFACE_SIDE_STYLE('',(#13717));
#13719=SURFACE_STYLE_USAGE(.BOTH.,#13718);
#13720=PRESENTATION_STYLE_ASSIGNMENT((#13719));
ENDSEC;
END-ISO-10303-21;
